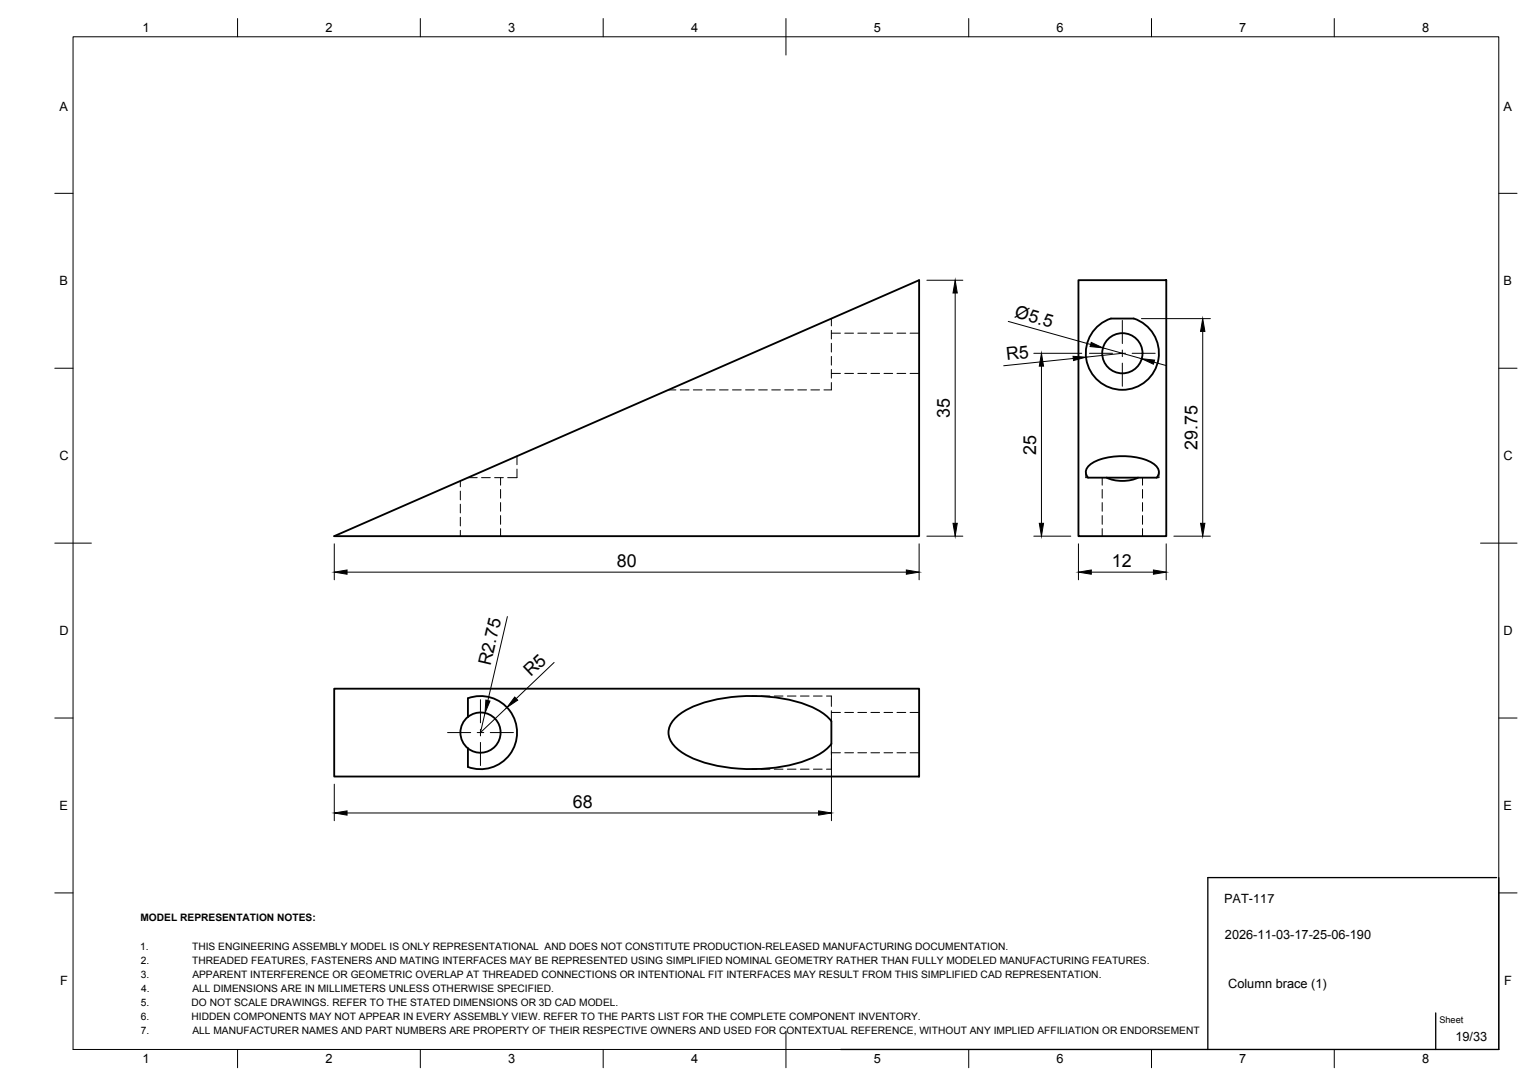
ISO-10303-21;
HEADER;
/* Generated by software containing ST-Developer
 * from STEP Tools, Inc. (www.steptools.com) 
 */

FILE_DESCRIPTION(
/* description */ ('Counterbalanced vertical column'),
/* implementation_level */ '2;1');

FILE_NAME(
/* name */ 'Column brace (1).step',
/* time_stamp */ '2026-10-29T16:47:22-07:00',
/* author */ (''),
/* organization */ (''),
/* preprocessor_version */ 'ST-DEVELOPER v20.2',
/* originating_system */ 'Autodesk Translation Framework v15.17.0.0',
/* authorisation */ '');

FILE_SCHEMA (('AUTOMOTIVE_DESIGN { 1 0 10303 214 3 1 1 }'));
ENDSEC;

DATA;
#10=MECHANICAL_DESIGN_GEOMETRIC_PRESENTATION_REPRESENTATION('',(#366),#15040);
#273=ELLIPSE('',#7732,0.545757787392906,0.5);
#274=ELLIPSE('',#7738,1.24744637118378,0.5);
#275=ELLIPSE('',#7739,0.300166783066098,0.275);
#296=SHAPE_REPRESENTATION_RELATIONSHIP('SRR','None',#15200,#331);
#331=ADVANCED_BREP_SHAPE_REPRESENTATION('',(#401),#15019);
#366=STYLED_ITEM('',(#15471),#401);
#401=MANIFOLD_SOLID_BREP('Body1',#7089);
#473=FACE_BOUND('',#1416,.T.);
#474=FACE_BOUND('',#1417,.T.);
#475=FACE_BOUND('',#1420,.T.);
#476=FACE_BOUND('',#1424,.T.);
#477=FACE_BOUND('',#1426,.T.);
#612=PLANE('',#7734);
#613=PLANE('',#7737);
#614=PLANE('',#7742);
#615=PLANE('',#7748);
#616=PLANE('',#7749);
#617=PLANE('',#7750);
#618=PLANE('',#7751);
#951=FACE_OUTER_BOUND('',#1413,.T.);
#952=FACE_OUTER_BOUND('',#1414,.T.);
#953=FACE_OUTER_BOUND('',#1415,.T.);
#954=FACE_OUTER_BOUND('',#1418,.T.);
#955=FACE_OUTER_BOUND('',#1419,.T.);
#956=FACE_OUTER_BOUND('',#1421,.T.);
#957=FACE_OUTER_BOUND('',#1422,.T.);
#958=FACE_OUTER_BOUND('',#1423,.T.);
#959=FACE_OUTER_BOUND('',#1425,.T.);
#960=FACE_OUTER_BOUND('',#1427,.T.);
#961=FACE_OUTER_BOUND('',#1428,.T.);
#1413=EDGE_LOOP('',(#5268,#5269));
#1414=EDGE_LOOP('',(#5270,#5271,#5272,#5273,#5274));
#1415=EDGE_LOOP('',(#5275,#5276,#5277,#5278));
#1416=EDGE_LOOP('',(#5279,#5280));
#1417=EDGE_LOOP('',(#5281,#5282,#5283,#5284));
#1418=EDGE_LOOP('',(#5285,#5286,#5287,#5288,#5289,#5290));
#1419=EDGE_LOOP('',(#5291,#5292));
#1420=EDGE_LOOP('',(#5293));
#1421=EDGE_LOOP('',(#5294,#5295));
#1422=EDGE_LOOP('',(#5296,#5297,#5298,#5299));
#1423=EDGE_LOOP('',(#5300,#5301,#5302,#5303));
#1424=EDGE_LOOP('',(#5304));
#1425=EDGE_LOOP('',(#5305,#5306,#5307,#5308));
#1426=EDGE_LOOP('',(#5309));
#1427=EDGE_LOOP('',(#5310,#5311,#5312));
#1428=EDGE_LOOP('',(#5313,#5314,#5315));
#1900=LINE('',#13527,#2571);
#1901=LINE('',#13532,#2572);
#1902=LINE('',#13536,#2573);
#1903=LINE('',#13538,#2574);
#1904=LINE('',#13540,#2575);
#1905=LINE('',#13541,#2576);
#1906=LINE('',#13545,#2577);
#1907=LINE('',#13550,#2578);
#1908=LINE('',#13559,#2579);
#1909=LINE('',#13562,#2580);
#1910=LINE('',#13564,#2581);
#1911=LINE('',#13565,#2582);
#1912=LINE('',#13567,#2583);
#1913=LINE('',#13568,#2584);
#2571=VECTOR('',#8844,1.);
#2572=VECTOR('',#8849,1.);
#2573=VECTOR('',#8852,1.);
#2574=VECTOR('',#8853,1.);
#2575=VECTOR('',#8854,1.);
#2576=VECTOR('',#8855,1.);
#2577=VECTOR('',#8858,1.);
#2578=VECTOR('',#8865,0.275);
#2579=VECTOR('',#8878,0.275);
#2580=VECTOR('',#8881,1.);
#2581=VECTOR('',#8882,1.);
#2582=VECTOR('',#8883,1.);
#2583=VECTOR('',#8886,1.);
#2584=VECTOR('',#8887,1.);
#3180=CIRCLE('',#7733,0.5);
#3181=CIRCLE('',#7735,0.275);
#3182=CIRCLE('',#7736,0.275);
#3183=CIRCLE('',#7741,0.275);
#3184=CIRCLE('',#7743,0.5);
#3185=CIRCLE('',#7744,0.275);
#3186=CIRCLE('',#7747,0.275);
#3466=VERTEX_POINT('',#13521);
#3467=VERTEX_POINT('',#13522);
#3468=VERTEX_POINT('',#13526);
#3469=VERTEX_POINT('',#13528);
#3470=VERTEX_POINT('',#13530);
#3471=VERTEX_POINT('',#13534);
#3472=VERTEX_POINT('',#13535);
#3473=VERTEX_POINT('',#13537);
#3474=VERTEX_POINT('',#13539);
#3475=VERTEX_POINT('',#13542);
#3476=VERTEX_POINT('',#13543);
#3477=VERTEX_POINT('',#13548);
#3478=VERTEX_POINT('',#13553);
#3479=VERTEX_POINT('',#13557);
#3480=VERTEX_POINT('',#13561);
#3481=VERTEX_POINT('',#13563);
#4135=EDGE_CURVE('',#3466,#3467,#273,.T.);
#4136=EDGE_CURVE('',#3467,#3466,#3180,.T.);
#4137=EDGE_CURVE('',#3468,#3466,#1900,.T.);
#4138=EDGE_CURVE('',#3469,#3468,#3181,.T.);
#4139=EDGE_CURVE('',#3470,#3469,#3182,.T.);
#4140=EDGE_CURVE('',#3467,#3470,#1901,.T.);
#4141=EDGE_CURVE('',#3471,#3472,#1902,.T.);
#4142=EDGE_CURVE('',#3472,#3473,#1903,.T.);
#4143=EDGE_CURVE('',#3474,#3473,#1904,.T.);
#4144=EDGE_CURVE('',#3471,#3474,#1905,.T.);
#4145=EDGE_CURVE('',#3475,#3476,#274,.T.);
#4146=EDGE_CURVE('',#3476,#3475,#1906,.T.);
#4147=EDGE_CURVE('',#3470,#3468,#275,.T.);
#4148=EDGE_CURVE('',#3477,#3477,#3183,.T.);
#4149=EDGE_CURVE('',#3477,#3469,#1907,.T.);
#4150=EDGE_CURVE('',#3476,#3475,#3184,.T.);
#4151=EDGE_CURVE('',#3478,#3478,#3185,.T.);
#4152=EDGE_CURVE('',#3479,#3479,#3186,.T.);
#4153=EDGE_CURVE('',#3479,#3478,#1908,.T.);
#4154=EDGE_CURVE('',#3480,#3471,#1909,.T.);
#4155=EDGE_CURVE('',#3481,#3474,#1910,.T.);
#4156=EDGE_CURVE('',#3480,#3481,#1911,.T.);
#4157=EDGE_CURVE('',#3472,#3480,#1912,.T.);
#4158=EDGE_CURVE('',#3473,#3481,#1913,.T.);
#5268=ORIENTED_EDGE('',*,*,#4135,.F.);
#5269=ORIENTED_EDGE('',*,*,#4136,.F.);
#5270=ORIENTED_EDGE('',*,*,#4137,.F.);
#5271=ORIENTED_EDGE('',*,*,#4138,.F.);
#5272=ORIENTED_EDGE('',*,*,#4139,.F.);
#5273=ORIENTED_EDGE('',*,*,#4140,.F.);
#5274=ORIENTED_EDGE('',*,*,#4136,.T.);
#5275=ORIENTED_EDGE('',*,*,#4141,.T.);
#5276=ORIENTED_EDGE('',*,*,#4142,.T.);
#5277=ORIENTED_EDGE('',*,*,#4143,.F.);
#5278=ORIENTED_EDGE('',*,*,#4144,.F.);
#5279=ORIENTED_EDGE('',*,*,#4145,.T.);
#5280=ORIENTED_EDGE('',*,*,#4146,.T.);
#5281=ORIENTED_EDGE('',*,*,#4137,.T.);
#5282=ORIENTED_EDGE('',*,*,#4135,.T.);
#5283=ORIENTED_EDGE('',*,*,#4140,.T.);
#5284=ORIENTED_EDGE('',*,*,#4147,.T.);
#5285=ORIENTED_EDGE('',*,*,#4148,.F.);
#5286=ORIENTED_EDGE('',*,*,#4149,.T.);
#5287=ORIENTED_EDGE('',*,*,#4138,.T.);
#5288=ORIENTED_EDGE('',*,*,#4147,.F.);
#5289=ORIENTED_EDGE('',*,*,#4139,.T.);
#5290=ORIENTED_EDGE('',*,*,#4149,.F.);
#5291=ORIENTED_EDGE('',*,*,#4146,.F.);
#5292=ORIENTED_EDGE('',*,*,#4150,.T.);
#5293=ORIENTED_EDGE('',*,*,#4151,.F.);
#5294=ORIENTED_EDGE('',*,*,#4145,.F.);
#5295=ORIENTED_EDGE('',*,*,#4150,.F.);
#5296=ORIENTED_EDGE('',*,*,#4152,.F.);
#5297=ORIENTED_EDGE('',*,*,#4153,.T.);
#5298=ORIENTED_EDGE('',*,*,#4151,.T.);
#5299=ORIENTED_EDGE('',*,*,#4153,.F.);
#5300=ORIENTED_EDGE('',*,*,#4154,.T.);
#5301=ORIENTED_EDGE('',*,*,#4144,.T.);
#5302=ORIENTED_EDGE('',*,*,#4155,.F.);
#5303=ORIENTED_EDGE('',*,*,#4156,.F.);
#5304=ORIENTED_EDGE('',*,*,#4152,.T.);
#5305=ORIENTED_EDGE('',*,*,#4157,.T.);
#5306=ORIENTED_EDGE('',*,*,#4156,.T.);
#5307=ORIENTED_EDGE('',*,*,#4158,.F.);
#5308=ORIENTED_EDGE('',*,*,#4142,.F.);
#5309=ORIENTED_EDGE('',*,*,#4148,.T.);
#5310=ORIENTED_EDGE('',*,*,#4158,.T.);
#5311=ORIENTED_EDGE('',*,*,#4155,.T.);
#5312=ORIENTED_EDGE('',*,*,#4143,.T.);
#5313=ORIENTED_EDGE('',*,*,#4157,.F.);
#5314=ORIENTED_EDGE('',*,*,#4141,.F.);
#5315=ORIENTED_EDGE('',*,*,#4154,.F.);
#6617=CYLINDRICAL_SURFACE('',#7731,0.5);
#6618=CYLINDRICAL_SURFACE('',#7740,0.275);
#6619=CYLINDRICAL_SURFACE('',#7745,0.5);
#6620=CYLINDRICAL_SURFACE('',#7746,0.275);
#6793=ADVANCED_FACE('',(#951),#6617,.F.);
#6794=ADVANCED_FACE('',(#952),#612,.T.);
#6795=ADVANCED_FACE('',(#953,#473,#474),#613,.T.);
#6796=ADVANCED_FACE('',(#954),#6618,.F.);
#6797=ADVANCED_FACE('',(#955,#475),#614,.T.);
#6798=ADVANCED_FACE('',(#956),#6619,.F.);
#6799=ADVANCED_FACE('',(#957),#6620,.F.);
#6800=ADVANCED_FACE('',(#958,#476),#615,.T.);
#6801=ADVANCED_FACE('',(#959,#477),#616,.T.);
#6802=ADVANCED_FACE('',(#960),#617,.T.);
#6803=ADVANCED_FACE('',(#961),#618,.F.);
#7089=CLOSED_SHELL('',(#6793,#6794,#6795,#6796,#6797,#6798,#6799,#6800,
#6801,#6802,#6803));
#7730=AXIS2_PLACEMENT_3D('',#13519,#8834,#8835);
#7731=AXIS2_PLACEMENT_3D('',#13520,#8836,#8837);
#7732=AXIS2_PLACEMENT_3D('',#13523,#8838,#8839);
#7733=AXIS2_PLACEMENT_3D('',#13524,#8840,#8841);
#7734=AXIS2_PLACEMENT_3D('',#13525,#8842,#8843);
#7735=AXIS2_PLACEMENT_3D('',#13529,#8845,#8846);
#7736=AXIS2_PLACEMENT_3D('',#13531,#8847,#8848);
#7737=AXIS2_PLACEMENT_3D('',#13533,#8850,#8851);
#7738=AXIS2_PLACEMENT_3D('',#13544,#8856,#8857);
#7739=AXIS2_PLACEMENT_3D('',#13546,#8859,#8860);
#7740=AXIS2_PLACEMENT_3D('',#13547,#8861,#8862);
#7741=AXIS2_PLACEMENT_3D('',#13549,#8863,#8864);
#7742=AXIS2_PLACEMENT_3D('',#13551,#8866,#8867);
#7743=AXIS2_PLACEMENT_3D('',#13552,#8868,#8869);
#7744=AXIS2_PLACEMENT_3D('',#13554,#8870,#8871);
#7745=AXIS2_PLACEMENT_3D('',#13555,#8872,#8873);
#7746=AXIS2_PLACEMENT_3D('',#13556,#8874,#8875);
#7747=AXIS2_PLACEMENT_3D('',#13558,#8876,#8877);
#7748=AXIS2_PLACEMENT_3D('',#13560,#8879,#8880);
#7749=AXIS2_PLACEMENT_3D('',#13566,#8884,#8885);
#7750=AXIS2_PLACEMENT_3D('',#13569,#8888,#8889);
#7751=AXIS2_PLACEMENT_3D('',#13570,#8890,#8891);
#8834=DIRECTION('axis',(0.,0.,1.));
#8835=DIRECTION('refdir',(1.,0.,0.));
#8836=DIRECTION('center_axis',(0.,1.,0.));
#8837=DIRECTION('ref_axis',(6.12323399573677E-17,0.,-1.));
#8838=DIRECTION('center_axis',(0.,-0.916157334902189,-0.400818834019708));
#8839=DIRECTION('ref_axis',(0.,0.400818834019708,-0.916157334902189));
#8840=DIRECTION('center_axis',(0.,1.,0.));
#8841=DIRECTION('ref_axis',(1.,0.,0.));
#8842=DIRECTION('center_axis',(0.,1.,0.));
#8843=DIRECTION('ref_axis',(1.,0.,0.));
#8844=DIRECTION('',(-1.,0.,0.));
#8845=DIRECTION('center_axis',(0.,1.,0.));
#8846=DIRECTION('ref_axis',(1.,0.,0.));
#8847=DIRECTION('center_axis',(0.,1.,0.));
#8848=DIRECTION('ref_axis',(1.,0.,0.));
#8849=DIRECTION('',(-1.,0.,0.));
#8850=DIRECTION('center_axis',(0.,0.916157334902189,0.400818834019708));
#8851=DIRECTION('ref_axis',(0.,-0.400818834019708,0.916157334902189));
#8852=DIRECTION('',(0.,-0.400818834019708,0.916157334902189));
#8853=DIRECTION('',(1.,0.,0.));
#8854=DIRECTION('',(0.,-0.400818834019708,0.916157334902189));
#8855=DIRECTION('',(1.,0.,0.));
#8856=DIRECTION('center_axis',(0.,-0.916157334902189,-0.400818834019708));
#8857=DIRECTION('ref_axis',(0.,0.400818834019708,-0.916157334902189));
#8858=DIRECTION('',(1.,0.,0.));
#8859=DIRECTION('center_axis',(0.,-0.916157334902189,-0.400818834019708));
#8860=DIRECTION('ref_axis',(0.,0.400818834019708,-0.916157334902189));
#8861=DIRECTION('center_axis',(0.,1.,0.));
#8862=DIRECTION('ref_axis',(1.,0.,0.));
#8863=DIRECTION('center_axis',(0.,1.,0.));
#8864=DIRECTION('ref_axis',(1.,0.,0.));
#8865=DIRECTION('',(0.,1.,0.));
#8866=DIRECTION('center_axis',(0.,0.,1.));
#8867=DIRECTION('ref_axis',(1.,0.,0.));
#8868=DIRECTION('center_axis',(0.,0.,1.));
#8869=DIRECTION('ref_axis',(1.,0.,0.));
#8870=DIRECTION('center_axis',(0.,0.,1.));
#8871=DIRECTION('ref_axis',(1.,0.,0.));
#8872=DIRECTION('center_axis',(0.,0.,1.));
#8873=DIRECTION('ref_axis',(-1.83697019872103E-16,-1.,0.));
#8874=DIRECTION('center_axis',(0.,0.,1.));
#8875=DIRECTION('ref_axis',(1.,0.,0.));
#8876=DIRECTION('center_axis',(0.,0.,1.));
#8877=DIRECTION('ref_axis',(1.,0.,0.));
#8878=DIRECTION('',(0.,0.,1.));
#8879=DIRECTION('center_axis',(0.,0.,-1.));
#8880=DIRECTION('ref_axis',(0.,1.,0.));
#8881=DIRECTION('',(0.,1.,0.));
#8882=DIRECTION('',(0.,1.,0.));
#8883=DIRECTION('',(1.,0.,0.));
#8884=DIRECTION('center_axis',(0.,-1.,0.));
#8885=DIRECTION('ref_axis',(0.,0.,-1.));
#8886=DIRECTION('',(0.,0.,-1.));
#8887=DIRECTION('',(0.,0.,-1.));
#8888=DIRECTION('center_axis',(1.,0.,0.));
#8889=DIRECTION('ref_axis',(0.,0.,-1.));
#8890=DIRECTION('center_axis',(1.,0.,0.));
#8891=DIRECTION('ref_axis',(0.,0.,-1.));
#13519=CARTESIAN_POINT('',(0.,0.,0.));
#13520=CARTESIAN_POINT('Origin',(3.,1.8,6.));
#13521=CARTESIAN_POINT('',(2.53030622220647,1.8,6.17142857142857));
#13522=CARTESIAN_POINT('',(3.46969377779353,1.8,6.17142857142857));
#13523=CARTESIAN_POINT('Origin',(3.,1.875,6.));
#13524=CARTESIAN_POINT('Origin',(3.,1.8,6.));
#13525=CARTESIAN_POINT('Origin',(3.,1.8,6.));
#13526=CARTESIAN_POINT('',(2.78497152537871,1.8,6.17142857142857));
#13527=CARTESIAN_POINT('',(2.7,1.8,6.17142857142857));
#13528=CARTESIAN_POINT('',(2.725,1.8,6.));
#13529=CARTESIAN_POINT('Origin',(3.,1.8,6.));
#13530=CARTESIAN_POINT('',(3.21502847462129,1.8,6.17142857142857));
#13531=CARTESIAN_POINT('Origin',(3.,1.8,6.));
#13532=CARTESIAN_POINT('',(2.7,1.8,6.17142857142857));
#13533=CARTESIAN_POINT('Origin',(2.4,4.5,0.));
#13534=CARTESIAN_POINT('',(2.4,4.5,0.));
#13535=CARTESIAN_POINT('',(2.4,1.,8.));
#13536=CARTESIAN_POINT('',(2.4,4.5,0.));
#13537=CARTESIAN_POINT('',(3.6,1.,8.));
#13538=CARTESIAN_POINT('',(2.4,1.,8.));
#13539=CARTESIAN_POINT('',(3.6,4.5,0.));
#13540=CARTESIAN_POINT('',(3.6,4.5,0.));
#13541=CARTESIAN_POINT('',(2.4,4.5,0.));
#13542=CARTESIAN_POINT('',(3.15612494995996,3.975,1.2));
#13543=CARTESIAN_POINT('',(2.84387505004004,3.975,1.2));
#13544=CARTESIAN_POINT('Origin',(3.,3.5,2.28571428571429));
#13545=CARTESIAN_POINT('',(2.7,3.975,1.2));
#13546=CARTESIAN_POINT('Origin',(3.,1.875,6.));
#13547=CARTESIAN_POINT('Origin',(3.,0.9,6.));
#13548=CARTESIAN_POINT('',(2.725,1.,6.));
#13549=CARTESIAN_POINT('Origin',(3.,1.,6.));
#13550=CARTESIAN_POINT('',(2.725,0.9,6.));
#13551=CARTESIAN_POINT('Origin',(3.,3.5,1.2));
#13552=CARTESIAN_POINT('Origin',(3.,3.5,1.2));
#13553=CARTESIAN_POINT('',(2.725,3.5,1.2));
#13554=CARTESIAN_POINT('Origin',(3.,3.5,1.2));
#13555=CARTESIAN_POINT('Origin',(3.,3.5,1.2));
#13556=CARTESIAN_POINT('Origin',(3.,3.5,-0.1));
#13557=CARTESIAN_POINT('',(2.725,3.5,0.));
#13558=CARTESIAN_POINT('Origin',(3.,3.5,0.));
#13559=CARTESIAN_POINT('',(2.725,3.5,-0.1));
#13560=CARTESIAN_POINT('Origin',(2.4,1.,0.));
#13561=CARTESIAN_POINT('',(2.4,1.,0.));
#13562=CARTESIAN_POINT('',(2.4,1.,0.));
#13563=CARTESIAN_POINT('',(3.6,1.,0.));
#13564=CARTESIAN_POINT('',(3.6,1.,0.));
#13565=CARTESIAN_POINT('',(2.4,1.,0.));
#13566=CARTESIAN_POINT('Origin',(2.4,1.,8.));
#13567=CARTESIAN_POINT('',(2.4,1.,8.));
#13568=CARTESIAN_POINT('',(3.6,1.,8.));
#13569=CARTESIAN_POINT('Origin',(3.6,2.75,4.));
#13570=CARTESIAN_POINT('Origin',(2.4,2.75,4.));
#14979=UNCERTAINTY_MEASURE_WITH_UNIT(LENGTH_MEASURE(0.001),#15041,
'DISTANCE_ACCURACY_VALUE',
'Maximum model space distance between geometric entities at asserted c
onnectivities');
#15000=UNCERTAINTY_MEASURE_WITH_UNIT(LENGTH_MEASURE(0.001),#15041,
'DISTANCE_ACCURACY_VALUE',
'Maximum model space distance between geometric entities at asserted c
onnectivities');
#15019=(
GEOMETRIC_REPRESENTATION_CONTEXT(3)
GLOBAL_UNCERTAINTY_ASSIGNED_CONTEXT((#14979))
GLOBAL_UNIT_ASSIGNED_CONTEXT((#15041,#15043,#15044))
REPRESENTATION_CONTEXT('','3D')
);
#15040=(
GEOMETRIC_REPRESENTATION_CONTEXT(3)
GLOBAL_UNCERTAINTY_ASSIGNED_CONTEXT((#15000))
GLOBAL_UNIT_ASSIGNED_CONTEXT((#15041,#15043,#15044))
REPRESENTATION_CONTEXT('','3D')
);
#15041=(
LENGTH_UNIT()
NAMED_UNIT(*)
SI_UNIT(.CENTI.,.METRE.)
);
#15043=(
NAMED_UNIT(*)
PLANE_ANGLE_UNIT()
SI_UNIT($,.RADIAN.)
);
#15044=(
NAMED_UNIT(*)
SI_UNIT($,.STERADIAN.)
SOLID_ANGLE_UNIT()
);
#15063=SHAPE_DEFINITION_REPRESENTATION(#15102,#15200);
#15102=PRODUCT_DEFINITION_SHAPE('',$,#15240);
#15200=SHAPE_REPRESENTATION('',(#7730),#15019);
#15221=PRODUCT_DEFINITION_CONTEXT('part definition',#15340,'design');
#15240=PRODUCT_DEFINITION('Column brace (1)','Column brace (1)',#15279,#15221);
#15279=PRODUCT_DEFINITION_FORMATION('',$,#15360);
#15340=APPLICATION_CONTEXT(
'Core Data for Automotive Mechanical Design Process');
#15341=PRODUCT_CONTEXT('part definition',#15340,'mechanical');
#15360=PRODUCT('Column brace (1)','Column brace (1)','Column brace (1)',(#15341));
#15465=COLOUR_RGB('Off White',0.89,0.88,0.83);
#15466=FILL_AREA_STYLE_COLOUR('',#15465);
#15467=FILL_AREA_STYLE('',(#15466));
#15468=SURFACE_STYLE_FILL_AREA(#15467);
#15469=SURFACE_SIDE_STYLE('',(#15468));
#15470=SURFACE_STYLE_USAGE(.BOTH.,#15469);
#15471=PRESENTATION_STYLE_ASSIGNMENT((#15470));
ENDSEC;
END-ISO-10303-21;
